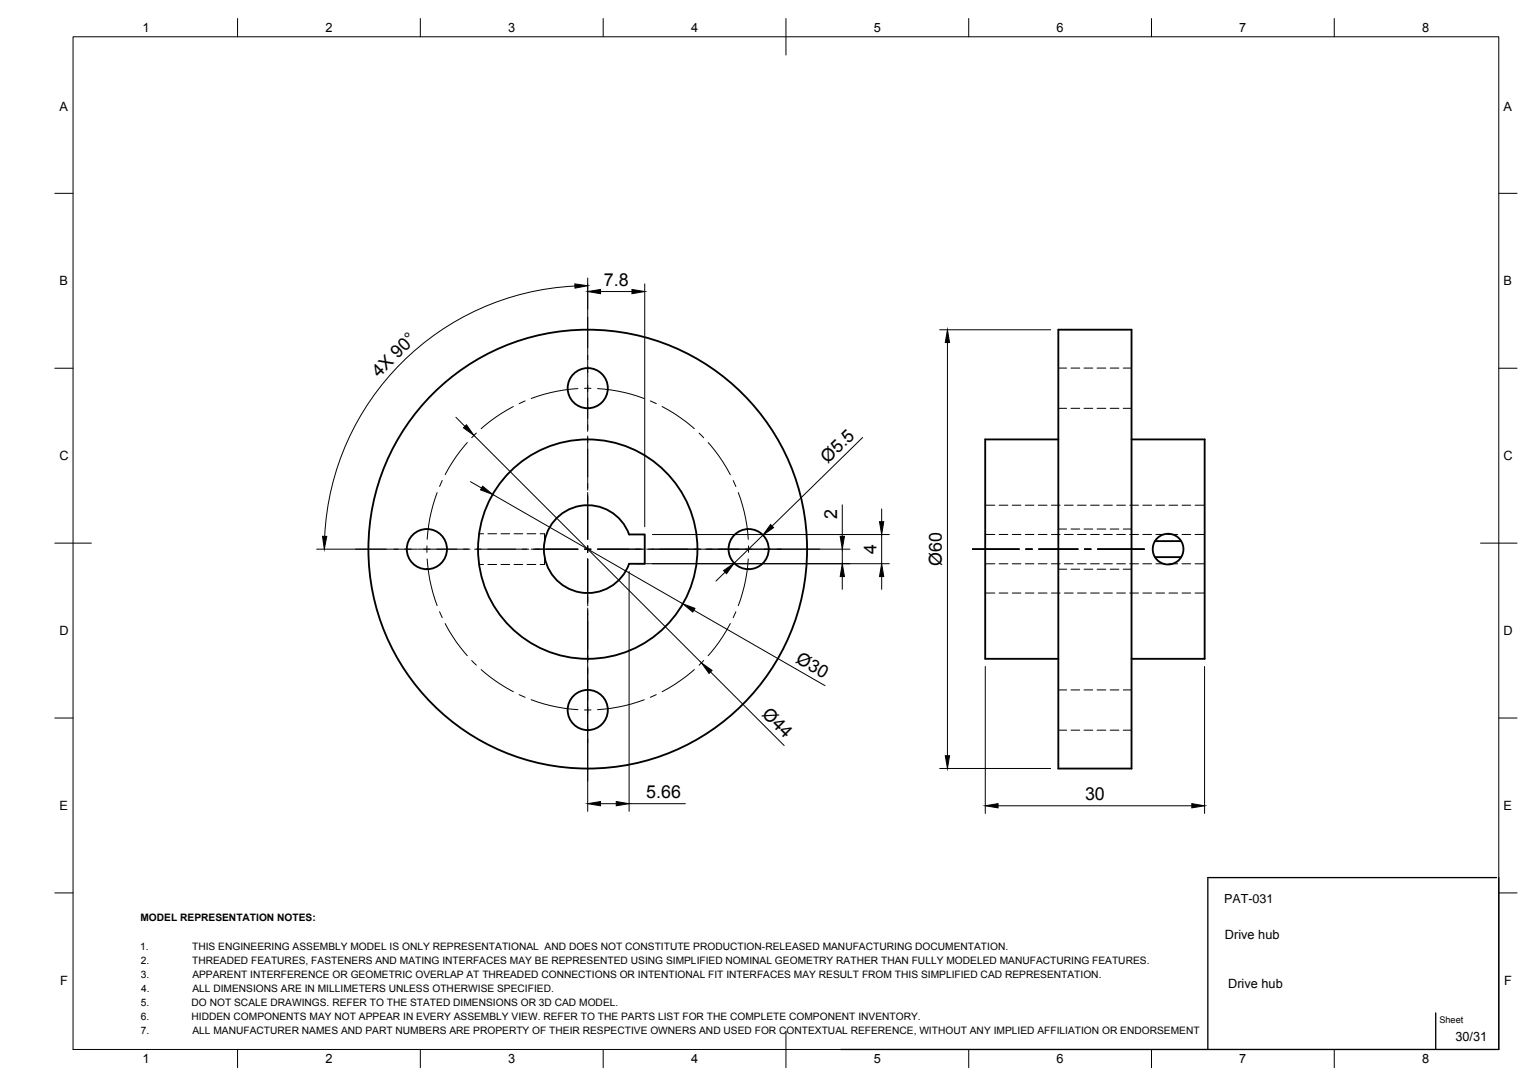
ISO-10303-21;
HEADER;
/* Generated by software containing ST-Developer
 * from STEP Tools, Inc. (www.steptools.com) 
 */

FILE_DESCRIPTION(
/* description */ ('Double-row support with tensioned shaft'),
/* implementation_level */ '2;1');

FILE_NAME(
/* name */ 'Drive hub.step',
/* time_stamp */ '2026-10-27T10:50:35-07:00',
/* author */ (''),
/* organization */ (''),
/* preprocessor_version */ 'ST-DEVELOPER v20.2',
/* originating_system */ 'Autodesk Translation Framework v15.17.0.0',
/* authorisation */ '');

FILE_SCHEMA (('AUTOMOTIVE_DESIGN { 1 0 10303 214 3 1 1 }'));
ENDSEC;

DATA;
#10=MECHANICAL_DESIGN_GEOMETRIC_PRESENTATION_REPRESENTATION('',(#509),#11559);
#387=B_SPLINE_CURVE_WITH_KNOTS('',3,(#11236,#11237,#11238,#11239,#11240,
#11241,#11242,#11243,#11244,#11245),.UNSPECIFIED.,.F.,.F.,(4,2,2,2,4),(0.847831445683411,
0.878274576930949,0.958092875386315,1.03791117384168,1.06835430508922),
 .UNSPECIFIED.);
#388=B_SPLINE_CURVE_WITH_KNOTS('',3,(#11251,#11252,#11253,#11254,#11255,
#11256,#11257,#11258,#11259,#11260,#11261,#11262,#11263,#11264,#11265,#11266,
#11267,#11268),.UNSPECIFIED.,.F.,.F.,(4,2,2,2,2,2,2,2,4),(0.,0.0792165807733633,
0.158433161546727,0.237648697074571,0.316864232602415,0.396079768130259,
0.475295303658103,0.554511884431466,0.63372846520483),.UNSPECIFIED.);
#389=B_SPLINE_CURVE_WITH_KNOTS('',3,(#11269,#11270,#11271,#11272,#11273,
#11274,#11275,#11276,#11277,#11278,#11279,#11280,#11281,#11282,#11283,#11284,
#11285,#11286),.UNSPECIFIED.,.F.,.F.,(4,2,2,2,2,2,2,2,4),(0.63372846520483,
0.712945045978193,0.792161626751556,0.8713771622794,0.950592697807245,1.02980823333509,
1.10902376886293,1.1882403496363,1.26745693040966),.UNSPECIFIED.);
#390=B_SPLINE_CURVE_WITH_KNOTS('',3,(#11289,#11290,#11291,#11292,#11293,
#11294,#11295,#11296,#11297,#11298),.UNSPECIFIED.,.F.,.F.,(4,2,2,2,4),(0.209102862092535,
0.239545993340072,0.319364291795438,0.399182590250804,0.429625721498342),
 .UNSPECIFIED.);
#444=SHAPE_REPRESENTATION_RELATIONSHIP('SRR','None',#11754,#476);
#476=ADVANCED_BREP_SHAPE_REPRESENTATION('',(#539),#11556);
#509=STYLED_ITEM('',(#11953),#539);
#539=MANIFOLD_SOLID_BREP('Body1',#6357);
#664=FACE_BOUND('',#1694,.T.);
#665=FACE_BOUND('',#1696,.T.);
#666=FACE_BOUND('',#1702,.T.);
#667=FACE_BOUND('',#1703,.T.);
#668=FACE_BOUND('',#1704,.T.);
#669=FACE_BOUND('',#1705,.T.);
#670=FACE_BOUND('',#1706,.T.);
#671=FACE_BOUND('',#1708,.T.);
#672=FACE_BOUND('',#1709,.T.);
#673=FACE_BOUND('',#1710,.T.);
#674=FACE_BOUND('',#1711,.T.);
#675=FACE_BOUND('',#1712,.T.);
#676=FACE_BOUND('',#1715,.T.);
#677=FACE_BOUND('',#1718,.T.);
#889=PLANE('',#7296);
#890=PLANE('',#7301);
#891=PLANE('',#7302);
#892=PLANE('',#7303);
#893=PLANE('',#7304);
#894=PLANE('',#7305);
#895=PLANE('',#7322);
#896=PLANE('',#7325);
#897=PLANE('',#7332);
#1221=FACE_OUTER_BOUND('',#1687,.T.);
#1222=FACE_OUTER_BOUND('',#1688,.T.);
#1223=FACE_OUTER_BOUND('',#1689,.T.);
#1224=FACE_OUTER_BOUND('',#1690,.T.);
#1225=FACE_OUTER_BOUND('',#1691,.T.);
#1226=FACE_OUTER_BOUND('',#1692,.T.);
#1227=FACE_OUTER_BOUND('',#1693,.T.);
#1228=FACE_OUTER_BOUND('',#1695,.T.);
#1229=FACE_OUTER_BOUND('',#1697,.T.);
#1230=FACE_OUTER_BOUND('',#1698,.T.);
#1231=FACE_OUTER_BOUND('',#1699,.T.);
#1232=FACE_OUTER_BOUND('',#1700,.T.);
#1233=FACE_OUTER_BOUND('',#1701,.T.);
#1234=FACE_OUTER_BOUND('',#1707,.T.);
#1235=FACE_OUTER_BOUND('',#1713,.T.);
#1236=FACE_OUTER_BOUND('',#1714,.T.);
#1237=FACE_OUTER_BOUND('',#1716,.T.);
#1238=FACE_OUTER_BOUND('',#1717,.T.);
#1687=EDGE_LOOP('',(#5706,#5707));
#1688=EDGE_LOOP('',(#5708,#5709,#5710,#5711,#5712,#5713,#5714,#5715,#5716));
#1689=EDGE_LOOP('',(#5717,#5718,#5719));
#1690=EDGE_LOOP('',(#5720,#5721,#5722,#5723));
#1691=EDGE_LOOP('',(#5724,#5725,#5726,#5727));
#1692=EDGE_LOOP('',(#5728,#5729,#5730,#5731));
#1693=EDGE_LOOP('',(#5732));
#1694=EDGE_LOOP('',(#5733,#5734,#5735,#5736));
#1695=EDGE_LOOP('',(#5737,#5738,#5739,#5740));
#1696=EDGE_LOOP('',(#5741,#5742,#5743,#5744));
#1697=EDGE_LOOP('',(#5745,#5746,#5747,#5748));
#1698=EDGE_LOOP('',(#5749,#5750,#5751,#5752));
#1699=EDGE_LOOP('',(#5753,#5754,#5755,#5756));
#1700=EDGE_LOOP('',(#5757,#5758,#5759,#5760));
#1701=EDGE_LOOP('',(#5761));
#1702=EDGE_LOOP('',(#5762));
#1703=EDGE_LOOP('',(#5763));
#1704=EDGE_LOOP('',(#5764));
#1705=EDGE_LOOP('',(#5765));
#1706=EDGE_LOOP('',(#5766));
#1707=EDGE_LOOP('',(#5767));
#1708=EDGE_LOOP('',(#5768));
#1709=EDGE_LOOP('',(#5769));
#1710=EDGE_LOOP('',(#5770));
#1711=EDGE_LOOP('',(#5771));
#1712=EDGE_LOOP('',(#5772));
#1713=EDGE_LOOP('',(#5773,#5774,#5775,#5776));
#1714=EDGE_LOOP('',(#5777,#5778,#5779,#5780));
#1715=EDGE_LOOP('',(#5781,#5782));
#1716=EDGE_LOOP('',(#5783,#5784,#5785,#5786));
#1717=EDGE_LOOP('',(#5787));
#1718=EDGE_LOOP('',(#5788,#5789,#5790,#5791));
#2224=LINE('',#11232,#2771);
#2225=LINE('',#11249,#2772);
#2226=LINE('',#11300,#2773);
#2227=LINE('',#11304,#2774);
#2228=LINE('',#11306,#2775);
#2229=LINE('',#11308,#2776);
#2230=LINE('',#11309,#2777);
#2231=LINE('',#11312,#2778);
#2232=LINE('',#11314,#2779);
#2233=LINE('',#11315,#2780);
#2234=LINE('',#11318,#2781);
#2235=LINE('',#11320,#2782);
#2236=LINE('',#11321,#2783);
#2237=LINE('',#11332,#2784);
#2238=LINE('',#11338,#2785);
#2239=LINE('',#11344,#2786);
#2240=LINE('',#11350,#2787);
#2241=LINE('',#11363,#2788);
#2242=LINE('',#11366,#2789);
#2243=LINE('',#11369,#2790);
#2771=VECTOR('',#9021,1.);
#2772=VECTOR('',#9028,0.21);
#2773=VECTOR('',#9033,1.);
#2774=VECTOR('',#9036,1.);
#2775=VECTOR('',#9037,1.);
#2776=VECTOR('',#9038,1.);
#2777=VECTOR('',#9039,1.);
#2778=VECTOR('',#9042,1.);
#2779=VECTOR('',#9043,1.);
#2780=VECTOR('',#9044,1.);
#2781=VECTOR('',#9047,1.);
#2782=VECTOR('',#9048,1.);
#2783=VECTOR('',#9049,1.);
#2784=VECTOR('',#9064,0.275);
#2785=VECTOR('',#9071,0.275);
#2786=VECTOR('',#9078,0.275);
#2787=VECTOR('',#9085,0.275);
#2788=VECTOR('',#9102,3.);
#2789=VECTOR('',#9105,1.5);
#2790=VECTOR('',#9110,1.5);
#3004=CIRCLE('',#7297,0.21);
#3005=CIRCLE('',#7299,0.21);
#3006=CIRCLE('',#7300,0.21);
#3007=CIRCLE('',#7306,1.5);
#3008=CIRCLE('',#7307,0.6);
#3009=CIRCLE('',#7309,0.6);
#3010=CIRCLE('',#7311,0.275);
#3011=CIRCLE('',#7312,0.275);
#3012=CIRCLE('',#7314,0.275);
#3013=CIRCLE('',#7315,0.275);
#3014=CIRCLE('',#7317,0.275);
#3015=CIRCLE('',#7318,0.275);
#3016=CIRCLE('',#7320,0.275);
#3017=CIRCLE('',#7321,0.275);
#3018=CIRCLE('',#7323,3.);
#3019=CIRCLE('',#7324,1.5);
#3020=CIRCLE('',#7326,3.);
#3021=CIRCLE('',#7327,1.5);
#3022=CIRCLE('',#7330,1.5);
#3489=VERTEX_POINT('',#11230);
#3490=VERTEX_POINT('',#11231);
#3491=VERTEX_POINT('',#11235);
#3492=VERTEX_POINT('',#11246);
#3493=VERTEX_POINT('',#11248);
#3494=VERTEX_POINT('',#11250);
#3495=VERTEX_POINT('',#11287);
#3496=VERTEX_POINT('',#11302);
#3497=VERTEX_POINT('',#11303);
#3498=VERTEX_POINT('',#11305);
#3499=VERTEX_POINT('',#11307);
#3500=VERTEX_POINT('',#11311);
#3501=VERTEX_POINT('',#11313);
#3502=VERTEX_POINT('',#11317);
#3503=VERTEX_POINT('',#11319);
#3504=VERTEX_POINT('',#11323);
#3505=VERTEX_POINT('',#11329);
#3506=VERTEX_POINT('',#11331);
#3507=VERTEX_POINT('',#11335);
#3508=VERTEX_POINT('',#11337);
#3509=VERTEX_POINT('',#11341);
#3510=VERTEX_POINT('',#11343);
#3511=VERTEX_POINT('',#11347);
#3512=VERTEX_POINT('',#11349);
#3513=VERTEX_POINT('',#11353);
#3514=VERTEX_POINT('',#11355);
#3515=VERTEX_POINT('',#11358);
#3516=VERTEX_POINT('',#11360);
#3517=VERTEX_POINT('',#11365);
#4238=EDGE_CURVE('',#3489,#3490,#2224,.T.);
#4239=EDGE_CURVE('',#3489,#3490,#3004,.T.);
#4240=EDGE_CURVE('',#3491,#3489,#387,.T.);
#4241=EDGE_CURVE('',#3492,#3491,#3005,.T.);
#4242=EDGE_CURVE('',#3492,#3493,#2225,.T.);
#4243=EDGE_CURVE('',#3494,#3493,#388,.T.);
#4244=EDGE_CURVE('',#3493,#3494,#389,.T.);
#4245=EDGE_CURVE('',#3495,#3492,#3006,.T.);
#4246=EDGE_CURVE('',#3490,#3495,#390,.T.);
#4247=EDGE_CURVE('',#3495,#3491,#2226,.T.);
#4248=EDGE_CURVE('',#3496,#3497,#2227,.T.);
#4249=EDGE_CURVE('',#3496,#3498,#2228,.T.);
#4250=EDGE_CURVE('',#3499,#3498,#2229,.T.);
#4251=EDGE_CURVE('',#3497,#3499,#2230,.T.);
#4252=EDGE_CURVE('',#3500,#3496,#2231,.T.);
#4253=EDGE_CURVE('',#3500,#3501,#2232,.T.);
#4254=EDGE_CURVE('',#3498,#3501,#2233,.T.);
#4255=EDGE_CURVE('',#3502,#3500,#2234,.T.);
#4256=EDGE_CURVE('',#3503,#3502,#2235,.T.);
#4257=EDGE_CURVE('',#3501,#3503,#2236,.T.);
#4258=EDGE_CURVE('',#3504,#3504,#3007,.T.);
#4259=EDGE_CURVE('',#3503,#3499,#3008,.T.);
#4260=EDGE_CURVE('',#3502,#3497,#3009,.T.);
#4261=EDGE_CURVE('',#3505,#3505,#3010,.T.);
#4262=EDGE_CURVE('',#3505,#3506,#2237,.T.);
#4263=EDGE_CURVE('',#3506,#3506,#3011,.T.);
#4264=EDGE_CURVE('',#3507,#3507,#3012,.T.);
#4265=EDGE_CURVE('',#3507,#3508,#2238,.T.);
#4266=EDGE_CURVE('',#3508,#3508,#3013,.T.);
#4267=EDGE_CURVE('',#3509,#3509,#3014,.T.);
#4268=EDGE_CURVE('',#3509,#3510,#2239,.T.);
#4269=EDGE_CURVE('',#3510,#3510,#3015,.T.);
#4270=EDGE_CURVE('',#3511,#3511,#3016,.T.);
#4271=EDGE_CURVE('',#3511,#3512,#2240,.T.);
#4272=EDGE_CURVE('',#3512,#3512,#3017,.T.);
#4273=EDGE_CURVE('',#3513,#3513,#3018,.T.);
#4274=EDGE_CURVE('',#3514,#3514,#3019,.T.);
#4275=EDGE_CURVE('',#3515,#3515,#3020,.T.);
#4276=EDGE_CURVE('',#3516,#3516,#3021,.T.);
#4277=EDGE_CURVE('',#3513,#3515,#2241,.T.);
#4278=EDGE_CURVE('',#3516,#3517,#2242,.T.);
#4279=EDGE_CURVE('',#3517,#3517,#3022,.T.);
#4280=EDGE_CURVE('',#3504,#3514,#2243,.T.);
#5706=ORIENTED_EDGE('',*,*,#4238,.F.);
#5707=ORIENTED_EDGE('',*,*,#4239,.T.);
#5708=ORIENTED_EDGE('',*,*,#4240,.F.);
#5709=ORIENTED_EDGE('',*,*,#4241,.F.);
#5710=ORIENTED_EDGE('',*,*,#4242,.T.);
#5711=ORIENTED_EDGE('',*,*,#4243,.F.);
#5712=ORIENTED_EDGE('',*,*,#4244,.F.);
#5713=ORIENTED_EDGE('',*,*,#4242,.F.);
#5714=ORIENTED_EDGE('',*,*,#4245,.F.);
#5715=ORIENTED_EDGE('',*,*,#4246,.F.);
#5716=ORIENTED_EDGE('',*,*,#4239,.F.);
#5717=ORIENTED_EDGE('',*,*,#4247,.F.);
#5718=ORIENTED_EDGE('',*,*,#4245,.T.);
#5719=ORIENTED_EDGE('',*,*,#4241,.T.);
#5720=ORIENTED_EDGE('',*,*,#4248,.F.);
#5721=ORIENTED_EDGE('',*,*,#4249,.T.);
#5722=ORIENTED_EDGE('',*,*,#4250,.F.);
#5723=ORIENTED_EDGE('',*,*,#4251,.F.);
#5724=ORIENTED_EDGE('',*,*,#4252,.F.);
#5725=ORIENTED_EDGE('',*,*,#4253,.T.);
#5726=ORIENTED_EDGE('',*,*,#4254,.F.);
#5727=ORIENTED_EDGE('',*,*,#4249,.F.);
#5728=ORIENTED_EDGE('',*,*,#4255,.F.);
#5729=ORIENTED_EDGE('',*,*,#4256,.F.);
#5730=ORIENTED_EDGE('',*,*,#4257,.F.);
#5731=ORIENTED_EDGE('',*,*,#4253,.F.);
#5732=ORIENTED_EDGE('',*,*,#4258,.T.);
#5733=ORIENTED_EDGE('',*,*,#4250,.T.);
#5734=ORIENTED_EDGE('',*,*,#4254,.T.);
#5735=ORIENTED_EDGE('',*,*,#4257,.T.);
#5736=ORIENTED_EDGE('',*,*,#4259,.T.);
#5737=ORIENTED_EDGE('',*,*,#4251,.T.);
#5738=ORIENTED_EDGE('',*,*,#4259,.F.);
#5739=ORIENTED_EDGE('',*,*,#4256,.T.);
#5740=ORIENTED_EDGE('',*,*,#4260,.T.);
#5741=ORIENTED_EDGE('',*,*,#4246,.T.);
#5742=ORIENTED_EDGE('',*,*,#4247,.T.);
#5743=ORIENTED_EDGE('',*,*,#4240,.T.);
#5744=ORIENTED_EDGE('',*,*,#4238,.T.);
#5745=ORIENTED_EDGE('',*,*,#4261,.F.);
#5746=ORIENTED_EDGE('',*,*,#4262,.T.);
#5747=ORIENTED_EDGE('',*,*,#4263,.F.);
#5748=ORIENTED_EDGE('',*,*,#4262,.F.);
#5749=ORIENTED_EDGE('',*,*,#4264,.F.);
#5750=ORIENTED_EDGE('',*,*,#4265,.T.);
#5751=ORIENTED_EDGE('',*,*,#4266,.F.);
#5752=ORIENTED_EDGE('',*,*,#4265,.F.);
#5753=ORIENTED_EDGE('',*,*,#4267,.F.);
#5754=ORIENTED_EDGE('',*,*,#4268,.T.);
#5755=ORIENTED_EDGE('',*,*,#4269,.F.);
#5756=ORIENTED_EDGE('',*,*,#4268,.F.);
#5757=ORIENTED_EDGE('',*,*,#4270,.F.);
#5758=ORIENTED_EDGE('',*,*,#4271,.T.);
#5759=ORIENTED_EDGE('',*,*,#4272,.F.);
#5760=ORIENTED_EDGE('',*,*,#4271,.F.);
#5761=ORIENTED_EDGE('',*,*,#4273,.T.);
#5762=ORIENTED_EDGE('',*,*,#4274,.F.);
#5763=ORIENTED_EDGE('',*,*,#4272,.T.);
#5764=ORIENTED_EDGE('',*,*,#4269,.T.);
#5765=ORIENTED_EDGE('',*,*,#4266,.T.);
#5766=ORIENTED_EDGE('',*,*,#4263,.T.);
#5767=ORIENTED_EDGE('',*,*,#4275,.F.);
#5768=ORIENTED_EDGE('',*,*,#4276,.F.);
#5769=ORIENTED_EDGE('',*,*,#4270,.T.);
#5770=ORIENTED_EDGE('',*,*,#4267,.T.);
#5771=ORIENTED_EDGE('',*,*,#4264,.T.);
#5772=ORIENTED_EDGE('',*,*,#4261,.T.);
#5773=ORIENTED_EDGE('',*,*,#4273,.F.);
#5774=ORIENTED_EDGE('',*,*,#4277,.T.);
#5775=ORIENTED_EDGE('',*,*,#4275,.T.);
#5776=ORIENTED_EDGE('',*,*,#4277,.F.);
#5777=ORIENTED_EDGE('',*,*,#4276,.T.);
#5778=ORIENTED_EDGE('',*,*,#4278,.T.);
#5779=ORIENTED_EDGE('',*,*,#4279,.T.);
#5780=ORIENTED_EDGE('',*,*,#4278,.F.);
#5781=ORIENTED_EDGE('',*,*,#4243,.T.);
#5782=ORIENTED_EDGE('',*,*,#4244,.T.);
#5783=ORIENTED_EDGE('',*,*,#4258,.F.);
#5784=ORIENTED_EDGE('',*,*,#4280,.T.);
#5785=ORIENTED_EDGE('',*,*,#4274,.T.);
#5786=ORIENTED_EDGE('',*,*,#4280,.F.);
#5787=ORIENTED_EDGE('',*,*,#4279,.F.);
#5788=ORIENTED_EDGE('',*,*,#4248,.T.);
#5789=ORIENTED_EDGE('',*,*,#4260,.F.);
#5790=ORIENTED_EDGE('',*,*,#4255,.T.);
#5791=ORIENTED_EDGE('',*,*,#4252,.T.);
#5970=CYLINDRICAL_SURFACE('',#7298,0.21);
#5971=CYLINDRICAL_SURFACE('',#7308,0.6);
#5972=CYLINDRICAL_SURFACE('',#7310,0.275);
#5973=CYLINDRICAL_SURFACE('',#7313,0.275);
#5974=CYLINDRICAL_SURFACE('',#7316,0.275);
#5975=CYLINDRICAL_SURFACE('',#7319,0.275);
#5976=CYLINDRICAL_SURFACE('',#7328,3.);
#5977=CYLINDRICAL_SURFACE('',#7329,1.5);
#5978=CYLINDRICAL_SURFACE('',#7331,1.5);
#6284=ADVANCED_FACE('',(#1221),#889,.T.);
#6285=ADVANCED_FACE('',(#1222),#5970,.F.);
#6286=ADVANCED_FACE('',(#1223),#890,.T.);
#6287=ADVANCED_FACE('',(#1224),#891,.F.);
#6288=ADVANCED_FACE('',(#1225),#892,.F.);
#6289=ADVANCED_FACE('',(#1226),#893,.F.);
#6290=ADVANCED_FACE('',(#1227,#664),#894,.T.);
#6291=ADVANCED_FACE('',(#1228,#665),#5971,.F.);
#6292=ADVANCED_FACE('',(#1229),#5972,.F.);
#6293=ADVANCED_FACE('',(#1230),#5973,.F.);
#6294=ADVANCED_FACE('',(#1231),#5974,.F.);
#6295=ADVANCED_FACE('',(#1232),#5975,.F.);
#6296=ADVANCED_FACE('',(#1233,#666,#667,#668,#669,#670),#895,.T.);
#6297=ADVANCED_FACE('',(#1234,#671,#672,#673,#674,#675),#896,.F.);
#6298=ADVANCED_FACE('',(#1235),#5976,.T.);
#6299=ADVANCED_FACE('',(#1236,#676),#5977,.T.);
#6300=ADVANCED_FACE('',(#1237),#5978,.T.);
#6301=ADVANCED_FACE('',(#1238,#677),#897,.F.);
#6357=CLOSED_SHELL('',(#6284,#6285,#6286,#6287,#6288,#6289,#6290,#6291,
#6292,#6293,#6294,#6295,#6296,#6297,#6298,#6299,#6300,#6301));
#7295=AXIS2_PLACEMENT_3D('',#11228,#9017,#9018);
#7296=AXIS2_PLACEMENT_3D('',#11229,#9019,#9020);
#7297=AXIS2_PLACEMENT_3D('',#11233,#9022,#9023);
#7298=AXIS2_PLACEMENT_3D('',#11234,#9024,#9025);
#7299=AXIS2_PLACEMENT_3D('',#11247,#9026,#9027);
#7300=AXIS2_PLACEMENT_3D('',#11288,#9029,#9030);
#7301=AXIS2_PLACEMENT_3D('',#11299,#9031,#9032);
#7302=AXIS2_PLACEMENT_3D('',#11301,#9034,#9035);
#7303=AXIS2_PLACEMENT_3D('',#11310,#9040,#9041);
#7304=AXIS2_PLACEMENT_3D('',#11316,#9045,#9046);
#7305=AXIS2_PLACEMENT_3D('',#11322,#9050,#9051);
#7306=AXIS2_PLACEMENT_3D('',#11324,#9052,#9053);
#7307=AXIS2_PLACEMENT_3D('',#11325,#9054,#9055);
#7308=AXIS2_PLACEMENT_3D('',#11326,#9056,#9057);
#7309=AXIS2_PLACEMENT_3D('',#11327,#9058,#9059);
#7310=AXIS2_PLACEMENT_3D('',#11328,#9060,#9061);
#7311=AXIS2_PLACEMENT_3D('',#11330,#9062,#9063);
#7312=AXIS2_PLACEMENT_3D('',#11333,#9065,#9066);
#7313=AXIS2_PLACEMENT_3D('',#11334,#9067,#9068);
#7314=AXIS2_PLACEMENT_3D('',#11336,#9069,#9070);
#7315=AXIS2_PLACEMENT_3D('',#11339,#9072,#9073);
#7316=AXIS2_PLACEMENT_3D('',#11340,#9074,#9075);
#7317=AXIS2_PLACEMENT_3D('',#11342,#9076,#9077);
#7318=AXIS2_PLACEMENT_3D('',#11345,#9079,#9080);
#7319=AXIS2_PLACEMENT_3D('',#11346,#9081,#9082);
#7320=AXIS2_PLACEMENT_3D('',#11348,#9083,#9084);
#7321=AXIS2_PLACEMENT_3D('',#11351,#9086,#9087);
#7322=AXIS2_PLACEMENT_3D('',#11352,#9088,#9089);
#7323=AXIS2_PLACEMENT_3D('',#11354,#9090,#9091);
#7324=AXIS2_PLACEMENT_3D('',#11356,#9092,#9093);
#7325=AXIS2_PLACEMENT_3D('',#11357,#9094,#9095);
#7326=AXIS2_PLACEMENT_3D('',#11359,#9096,#9097);
#7327=AXIS2_PLACEMENT_3D('',#11361,#9098,#9099);
#7328=AXIS2_PLACEMENT_3D('',#11362,#9100,#9101);
#7329=AXIS2_PLACEMENT_3D('',#11364,#9103,#9104);
#7330=AXIS2_PLACEMENT_3D('',#11367,#9106,#9107);
#7331=AXIS2_PLACEMENT_3D('',#11368,#9108,#9109);
#7332=AXIS2_PLACEMENT_3D('',#11370,#9111,#9112);
#9017=DIRECTION('axis',(0.,0.,1.));
#9018=DIRECTION('refdir',(1.,0.,0.));
#9019=DIRECTION('center_axis',(0.,0.,1.));
#9020=DIRECTION('ref_axis',(1.,0.,0.));
#9021=DIRECTION('',(0.,1.,0.));
#9022=DIRECTION('center_axis',(0.,0.,1.));
#9023=DIRECTION('ref_axis',(1.,0.,0.));
#9024=DIRECTION('center_axis',(0.,0.,1.));
#9025=DIRECTION('ref_axis',(1.,0.,0.));
#9026=DIRECTION('center_axis',(0.,0.,1.));
#9027=DIRECTION('ref_axis',(1.,0.,0.));
#9028=DIRECTION('',(0.,0.,1.));
#9029=DIRECTION('center_axis',(0.,0.,1.));
#9030=DIRECTION('ref_axis',(1.,0.,0.));
#9031=DIRECTION('center_axis',(0.,0.,1.));
#9032=DIRECTION('ref_axis',(1.,0.,0.));
#9033=DIRECTION('',(0.,-1.,0.));
#9034=DIRECTION('center_axis',(-1.,0.,0.));
#9035=DIRECTION('ref_axis',(0.,0.,1.));
#9036=DIRECTION('',(0.,0.,1.));
#9037=DIRECTION('',(0.,1.,0.));
#9038=DIRECTION('',(0.,0.,-1.));
#9039=DIRECTION('',(0.,1.,0.));
#9040=DIRECTION('center_axis',(0.,0.,-1.));
#9041=DIRECTION('ref_axis',(-1.,0.,0.));
#9042=DIRECTION('',(-1.,0.,0.));
#9043=DIRECTION('',(0.,1.,0.));
#9044=DIRECTION('',(1.,0.,0.));
#9045=DIRECTION('center_axis',(1.,0.,0.));
#9046=DIRECTION('ref_axis',(0.,0.,-1.));
#9047=DIRECTION('',(0.,0.,-1.));
#9048=DIRECTION('',(0.,-1.,0.));
#9049=DIRECTION('',(0.,0.,1.));
#9050=DIRECTION('center_axis',(0.,1.,0.));
#9051=DIRECTION('ref_axis',(1.,0.,0.));
#9052=DIRECTION('center_axis',(0.,1.,0.));
#9053=DIRECTION('ref_axis',(1.,0.,0.));
#9054=DIRECTION('center_axis',(0.,-1.,0.));
#9055=DIRECTION('ref_axis',(1.,0.,0.));
#9056=DIRECTION('center_axis',(0.,1.,0.));
#9057=DIRECTION('ref_axis',(-1.83697019872103E-16,0.,1.));
#9058=DIRECTION('center_axis',(0.,-1.,0.));
#9059=DIRECTION('ref_axis',(1.,0.,0.));
#9060=DIRECTION('center_axis',(0.,1.,0.));
#9061=DIRECTION('ref_axis',(1.,0.,0.));
#9062=DIRECTION('center_axis',(0.,1.,0.));
#9063=DIRECTION('ref_axis',(1.,0.,0.));
#9064=DIRECTION('',(0.,1.,0.));
#9065=DIRECTION('center_axis',(0.,-1.,0.));
#9066=DIRECTION('ref_axis',(1.,0.,0.));
#9067=DIRECTION('center_axis',(0.,1.,0.));
#9068=DIRECTION('ref_axis',(1.,0.,0.));
#9069=DIRECTION('center_axis',(0.,1.,0.));
#9070=DIRECTION('ref_axis',(1.,0.,0.));
#9071=DIRECTION('',(0.,1.,0.));
#9072=DIRECTION('center_axis',(0.,-1.,0.));
#9073=DIRECTION('ref_axis',(1.,0.,0.));
#9074=DIRECTION('center_axis',(0.,1.,0.));
#9075=DIRECTION('ref_axis',(1.,0.,0.));
#9076=DIRECTION('center_axis',(0.,1.,0.));
#9077=DIRECTION('ref_axis',(1.,0.,0.));
#9078=DIRECTION('',(0.,1.,0.));
#9079=DIRECTION('center_axis',(0.,-1.,0.));
#9080=DIRECTION('ref_axis',(1.,0.,0.));
#9081=DIRECTION('center_axis',(0.,1.,0.));
#9082=DIRECTION('ref_axis',(1.,0.,0.));
#9083=DIRECTION('center_axis',(0.,1.,0.));
#9084=DIRECTION('ref_axis',(1.,0.,0.));
#9085=DIRECTION('',(0.,1.,0.));
#9086=DIRECTION('center_axis',(0.,-1.,0.));
#9087=DIRECTION('ref_axis',(1.,0.,0.));
#9088=DIRECTION('center_axis',(0.,1.,0.));
#9089=DIRECTION('ref_axis',(1.,0.,0.));
#9090=DIRECTION('center_axis',(0.,1.,0.));
#9091=DIRECTION('ref_axis',(1.,0.,0.));
#9092=DIRECTION('center_axis',(0.,1.,0.));
#9093=DIRECTION('ref_axis',(1.,0.,0.));
#9094=DIRECTION('center_axis',(0.,1.,0.));
#9095=DIRECTION('ref_axis',(1.,0.,0.));
#9096=DIRECTION('center_axis',(0.,1.,0.));
#9097=DIRECTION('ref_axis',(1.,0.,0.));
#9098=DIRECTION('center_axis',(0.,-1.,0.));
#9099=DIRECTION('ref_axis',(1.,0.,0.));
#9100=DIRECTION('center_axis',(0.,1.,0.));
#9101=DIRECTION('ref_axis',(1.,0.,0.));
#9102=DIRECTION('',(0.,-1.,0.));
#9103=DIRECTION('center_axis',(0.,1.,0.));
#9104=DIRECTION('ref_axis',(1.,0.,0.));
#9105=DIRECTION('',(0.,-1.,0.));
#9106=DIRECTION('center_axis',(0.,1.,0.));
#9107=DIRECTION('ref_axis',(1.,0.,0.));
#9108=DIRECTION('center_axis',(0.,1.,0.));
#9109=DIRECTION('ref_axis',(1.,0.,0.));
#9110=DIRECTION('',(0.,-1.,0.));
#9111=DIRECTION('center_axis',(0.,1.,0.));
#9112=DIRECTION('ref_axis',(1.,0.,0.));
#11228=CARTESIAN_POINT('',(0.,0.,0.));
#11229=CARTESIAN_POINT('Origin',(0.,7.5,10.59));
#11230=CARTESIAN_POINT('',(0.109087121146348,7.32055641555073,10.59));
#11231=CARTESIAN_POINT('',(0.109087121146348,7.67944358444927,10.59));
#11232=CARTESIAN_POINT('',(0.109087121146348,7.,10.59));
#11233=CARTESIAN_POINT('Origin',(0.,7.5,10.59));
#11234=CARTESIAN_POINT('Origin',(0.,7.5,10.59));
#11235=CARTESIAN_POINT('',(-0.109087121146348,7.32055641555073,10.59));
#11236=CARTESIAN_POINT('Ctrl Pts',(-0.109087121146348,7.32055641555073,
10.59));
#11237=CARTESIAN_POINT('Ctrl Pts',(-0.100058962329427,7.31506802844783,
10.5916692472112));
#11238=CARTESIAN_POINT('Ctrl Pts',(-0.0905297208284634,7.31021510111871,
10.5932143633855));
#11239=CARTESIAN_POINT('Ctrl Pts',(-0.0548356965671431,7.29536302924048,
10.598057680137));
#11240=CARTESIAN_POINT('Ctrl Pts',(-0.026606099485122,7.29,10.6));
#11241=CARTESIAN_POINT('Ctrl Pts',(0.0266060994851219,7.29,10.6));
#11242=CARTESIAN_POINT('Ctrl Pts',(0.054835696567143,7.29536302924048,10.598057680137));
#11243=CARTESIAN_POINT('Ctrl Pts',(0.0905297208284634,7.31021510111871,
10.5932143633855));
#11244=CARTESIAN_POINT('Ctrl Pts',(0.100058962329428,7.31506802844783,10.5916692472112));
#11245=CARTESIAN_POINT('Ctrl Pts',(0.109087121146348,7.32055641555073,10.59));
#11246=CARTESIAN_POINT('',(-0.21,7.5,10.59));
#11247=CARTESIAN_POINT('Origin',(0.,7.5,10.59));
#11248=CARTESIAN_POINT('',(-0.21,7.5,11.4852272553384));
#11249=CARTESIAN_POINT('',(-0.21,7.5,10.59));
#11250=CARTESIAN_POINT('',(0.21,7.5,11.4852272553384));
#11251=CARTESIAN_POINT('Ctrl Pts',(0.21,7.5,11.4852272553384));
#11252=CARTESIAN_POINT('Ctrl Pts',(0.21,7.47359447307555,11.4852272553384));
#11253=CARTESIAN_POINT('Ctrl Pts',(0.204715737269596,7.44545292590929,11.4860041595441));
#11254=CARTESIAN_POINT('Ctrl Pts',(0.183273763036332,7.39372373109487,11.4888007328232));
#11255=CARTESIAN_POINT('Ctrl Pts',(0.167117923970394,7.37013307587204,11.4907789715758));
#11256=CARTESIAN_POINT('Ctrl Pts',(0.129867169887369,7.33288232178902,11.4944848114133));
#11257=CARTESIAN_POINT('Ctrl Pts',(0.106276408305765,7.31672628999865,11.4964545565713));
#11258=CARTESIAN_POINT('Ctrl Pts',(0.0545468514059003,7.29528417517378,
11.4992316551565));
#11259=CARTESIAN_POINT('Ctrl Pts',(0.0264051785092814,7.29,11.5));
#11260=CARTESIAN_POINT('Ctrl Pts',(-0.0264051785092814,7.29,11.5));
#11261=CARTESIAN_POINT('Ctrl Pts',(-0.0545468514059002,7.29528417517378,
11.4992316551565));
#11262=CARTESIAN_POINT('Ctrl Pts',(-0.106276408305765,7.31672628999865,
11.4964545565713));
#11263=CARTESIAN_POINT('Ctrl Pts',(-0.129867169887369,7.33288232178902,
11.4944848114133));
#11264=CARTESIAN_POINT('Ctrl Pts',(-0.167117923970394,7.37013307587204,
11.4907789715758));
#11265=CARTESIAN_POINT('Ctrl Pts',(-0.183273763036332,7.39372373109487,
11.4888007328232));
#11266=CARTESIAN_POINT('Ctrl Pts',(-0.204715737269596,7.44545292590929,
11.4860041595441));
#11267=CARTESIAN_POINT('Ctrl Pts',(-0.21,7.47359447307555,11.4852272553384));
#11268=CARTESIAN_POINT('Ctrl Pts',(-0.21,7.5,11.4852272553384));
#11269=CARTESIAN_POINT('Ctrl Pts',(-0.21,7.5,11.4852272553384));
#11270=CARTESIAN_POINT('Ctrl Pts',(-0.21,7.52640552692445,11.4852272553384));
#11271=CARTESIAN_POINT('Ctrl Pts',(-0.204715737269596,7.55454707409071,
11.4860041595441));
#11272=CARTESIAN_POINT('Ctrl Pts',(-0.183273763036332,7.60627626890513,
11.4888007328232));
#11273=CARTESIAN_POINT('Ctrl Pts',(-0.167117923970394,7.62986692412796,
11.4907789715758));
#11274=CARTESIAN_POINT('Ctrl Pts',(-0.129867169887369,7.66711767821098,
11.4944848114133));
#11275=CARTESIAN_POINT('Ctrl Pts',(-0.106276408305765,7.68327371000135,
11.4964545565713));
#11276=CARTESIAN_POINT('Ctrl Pts',(-0.0545468514059003,7.70471582482622,
11.4992316551565));
#11277=CARTESIAN_POINT('Ctrl Pts',(-0.0264051785092814,7.71,11.5));
#11278=CARTESIAN_POINT('Ctrl Pts',(0.0264051785092813,7.71,11.5));
#11279=CARTESIAN_POINT('Ctrl Pts',(0.0545468514059002,7.70471582482622,
11.4992316551565));
#11280=CARTESIAN_POINT('Ctrl Pts',(0.106276408305765,7.68327371000135,11.4964545565713));
#11281=CARTESIAN_POINT('Ctrl Pts',(0.129867169887369,7.66711767821098,11.4944848114133));
#11282=CARTESIAN_POINT('Ctrl Pts',(0.167117923970394,7.62986692412796,11.4907789715758));
#11283=CARTESIAN_POINT('Ctrl Pts',(0.183273763036332,7.60627626890513,11.4888007328232));
#11284=CARTESIAN_POINT('Ctrl Pts',(0.204715737269596,7.55454707409071,11.4860041595441));
#11285=CARTESIAN_POINT('Ctrl Pts',(0.21,7.52640552692445,11.4852272553384));
#11286=CARTESIAN_POINT('Ctrl Pts',(0.21,7.5,11.4852272553384));
#11287=CARTESIAN_POINT('',(-0.109087121146348,7.67944358444927,10.59));
#11288=CARTESIAN_POINT('Origin',(0.,7.5,10.59));
#11289=CARTESIAN_POINT('Ctrl Pts',(0.109087121146348,7.67944358444927,10.59));
#11290=CARTESIAN_POINT('Ctrl Pts',(0.100058962329428,7.68493197155217,10.5916692472112));
#11291=CARTESIAN_POINT('Ctrl Pts',(0.0905297208284629,7.68978489888129,
10.5932143633855));
#11292=CARTESIAN_POINT('Ctrl Pts',(0.054835696567143,7.70463697075952,10.598057680137));
#11293=CARTESIAN_POINT('Ctrl Pts',(0.026606099485122,7.71,10.6));
#11294=CARTESIAN_POINT('Ctrl Pts',(-0.0266060994851219,7.71,10.6));
#11295=CARTESIAN_POINT('Ctrl Pts',(-0.054835696567143,7.70463697075952,
10.598057680137));
#11296=CARTESIAN_POINT('Ctrl Pts',(-0.0905297208284633,7.68978489888129,
10.5932143633855));
#11297=CARTESIAN_POINT('Ctrl Pts',(-0.100058962329427,7.68493197155217,
10.5916692472112));
#11298=CARTESIAN_POINT('Ctrl Pts',(-0.109087121146348,7.67944358444927,
10.59));
#11299=CARTESIAN_POINT('Origin',(0.,7.5,10.59));
#11300=CARTESIAN_POINT('',(-0.109087121146348,7.,10.59));
#11301=CARTESIAN_POINT('Origin',(-0.2,6.9,9.22));
#11302=CARTESIAN_POINT('',(-0.2,7.,9.22));
#11303=CARTESIAN_POINT('',(-0.2,7.,9.43431457505076));
#11304=CARTESIAN_POINT('',(-0.2,7.,9.61));
#11305=CARTESIAN_POINT('',(-0.2,10.,9.22));
#11306=CARTESIAN_POINT('',(-0.2,6.9,9.22));
#11307=CARTESIAN_POINT('',(-0.2,10.,9.43431457505076));
#11308=CARTESIAN_POINT('',(-0.2,10.,9.61));
#11309=CARTESIAN_POINT('',(-0.2,7.,9.43431457505076));
#11310=CARTESIAN_POINT('Origin',(0.2,6.9,9.22));
#11311=CARTESIAN_POINT('',(0.2,7.,9.22));
#11312=CARTESIAN_POINT('',(0.1,7.,9.22));
#11313=CARTESIAN_POINT('',(0.2,10.,9.22));
#11314=CARTESIAN_POINT('',(0.2,6.9,9.22));
#11315=CARTESIAN_POINT('',(0.1,10.,9.22));
#11316=CARTESIAN_POINT('Origin',(0.2,6.9,10.));
#11317=CARTESIAN_POINT('',(0.2,7.,9.43431457505076));
#11318=CARTESIAN_POINT('',(0.2,7.,10.));
#11319=CARTESIAN_POINT('',(0.2,10.,9.43431457505076));
#11320=CARTESIAN_POINT('',(0.2,7.,9.43431457505076));
#11321=CARTESIAN_POINT('',(0.2,10.,10.));
#11322=CARTESIAN_POINT('Origin',(0.,10.,10.));
#11323=CARTESIAN_POINT('',(-1.5,10.,10.));
#11324=CARTESIAN_POINT('Origin',(0.,10.,10.));
#11325=CARTESIAN_POINT('Origin',(0.,10.,10.));
#11326=CARTESIAN_POINT('Origin',(0.,7.,10.));
#11327=CARTESIAN_POINT('Origin',(0.,7.,10.));
#11328=CARTESIAN_POINT('Origin',(-2.2,7.9,10.));
#11329=CARTESIAN_POINT('',(-2.475,8.,10.));
#11330=CARTESIAN_POINT('Origin',(-2.2,8.,10.));
#11331=CARTESIAN_POINT('',(-2.475,9.,10.));
#11332=CARTESIAN_POINT('',(-2.475,7.9,10.));
#11333=CARTESIAN_POINT('Origin',(-2.2,9.,10.));
#11334=CARTESIAN_POINT('Origin',(1.34711147906209E-16,7.9,12.2));
#11335=CARTESIAN_POINT('',(-0.275,8.,12.2));
#11336=CARTESIAN_POINT('Origin',(1.34711147906209E-16,8.,12.2));
#11337=CARTESIAN_POINT('',(-0.275,9.,12.2));
#11338=CARTESIAN_POINT('',(-0.275,7.9,12.2));
#11339=CARTESIAN_POINT('Origin',(1.34711147906209E-16,9.,12.2));
#11340=CARTESIAN_POINT('Origin',(2.2,7.9,10.));
#11341=CARTESIAN_POINT('',(1.925,8.,10.));
#11342=CARTESIAN_POINT('Origin',(2.2,8.,10.));
#11343=CARTESIAN_POINT('',(1.925,9.,10.));
#11344=CARTESIAN_POINT('',(1.925,7.9,10.));
#11345=CARTESIAN_POINT('Origin',(2.2,9.,10.));
#11346=CARTESIAN_POINT('Origin',(-4.04133443718627E-16,7.9,7.8));
#11347=CARTESIAN_POINT('',(-0.275,8.,7.8));
#11348=CARTESIAN_POINT('Origin',(-4.04133443718627E-16,8.,7.8));
#11349=CARTESIAN_POINT('',(-0.275,9.,7.8));
#11350=CARTESIAN_POINT('',(-0.275,7.9,7.8));
#11351=CARTESIAN_POINT('Origin',(-4.04133443718627E-16,9.,7.8));
#11352=CARTESIAN_POINT('Origin',(0.,9.,10.));
#11353=CARTESIAN_POINT('',(-3.,9.,10.));
#11354=CARTESIAN_POINT('Origin',(0.,9.,10.));
#11355=CARTESIAN_POINT('',(-1.5,9.,10.));
#11356=CARTESIAN_POINT('Origin',(0.,9.,10.));
#11357=CARTESIAN_POINT('Origin',(0.,8.,10.));
#11358=CARTESIAN_POINT('',(-3.,8.,10.));
#11359=CARTESIAN_POINT('Origin',(0.,8.,10.));
#11360=CARTESIAN_POINT('',(-1.5,8.,10.));
#11361=CARTESIAN_POINT('Origin',(0.,8.,10.));
#11362=CARTESIAN_POINT('Origin',(0.,8.,10.));
#11363=CARTESIAN_POINT('',(-3.,8.,10.));
#11364=CARTESIAN_POINT('Origin',(0.,7.,10.));
#11365=CARTESIAN_POINT('',(-1.5,7.,10.));
#11366=CARTESIAN_POINT('',(-1.5,7.,10.));
#11367=CARTESIAN_POINT('Origin',(0.,7.,10.));
#11368=CARTESIAN_POINT('Origin',(0.,7.,10.));
#11369=CARTESIAN_POINT('',(-1.5,7.,10.));
#11370=CARTESIAN_POINT('Origin',(0.,7.,10.));
#11519=UNCERTAINTY_MEASURE_WITH_UNIT(LENGTH_MEASURE(0.001),#11560,
'DISTANCE_ACCURACY_VALUE',
'Maximum model space distance between geometric entities at asserted c
onnectivities');
#11522=UNCERTAINTY_MEASURE_WITH_UNIT(LENGTH_MEASURE(0.001),#11560,
'DISTANCE_ACCURACY_VALUE',
'Maximum model space distance between geometric entities at asserted c
onnectivities');
#11556=(
GEOMETRIC_REPRESENTATION_CONTEXT(3)
GLOBAL_UNCERTAINTY_ASSIGNED_CONTEXT((#11519))
GLOBAL_UNIT_ASSIGNED_CONTEXT((#11560,#11562,#11563))
REPRESENTATION_CONTEXT('','3D')
);
#11559=(
GEOMETRIC_REPRESENTATION_CONTEXT(3)
GLOBAL_UNCERTAINTY_ASSIGNED_CONTEXT((#11522))
GLOBAL_UNIT_ASSIGNED_CONTEXT((#11560,#11562,#11563))
REPRESENTATION_CONTEXT('','3D')
);
#11560=(
LENGTH_UNIT()
NAMED_UNIT(*)
SI_UNIT(.CENTI.,.METRE.)
);
#11562=(
NAMED_UNIT(*)
PLANE_ANGLE_UNIT()
SI_UNIT($,.RADIAN.)
);
#11563=(
NAMED_UNIT(*)
SI_UNIT($,.STERADIAN.)
SOLID_ANGLE_UNIT()
);
#11597=SHAPE_DEFINITION_REPRESENTATION(#11708,#11754);
#11708=PRODUCT_DEFINITION_SHAPE('',$,#11791);
#11754=SHAPE_REPRESENTATION('',(#7295),#11556);
#11757=PRODUCT_DEFINITION_CONTEXT('part definition',#11867,'design');
#11791=PRODUCT_DEFINITION('Drive hub','Drive hub',#11827,#11757);
#11827=PRODUCT_DEFINITION_FORMATION('',$,#11902);
#11867=APPLICATION_CONTEXT(
'Core Data for Automotive Mechanical Design Process');
#11868=PRODUCT_CONTEXT('part definition',#11867,'mechanical');
#11902=PRODUCT('Drive hub','Drive hub','Drive hub',(#11868));
#11947=COLOUR_RGB('Light Blue',0.38,0.62,0.78);
#11948=FILL_AREA_STYLE_COLOUR('',#11947);
#11949=FILL_AREA_STYLE('',(#11948));
#11950=SURFACE_STYLE_FILL_AREA(#11949);
#11951=SURFACE_SIDE_STYLE('',(#11950));
#11952=SURFACE_STYLE_USAGE(.BOTH.,#11951);
#11953=PRESENTATION_STYLE_ASSIGNMENT((#11952));
ENDSEC;
END-ISO-10303-21;
